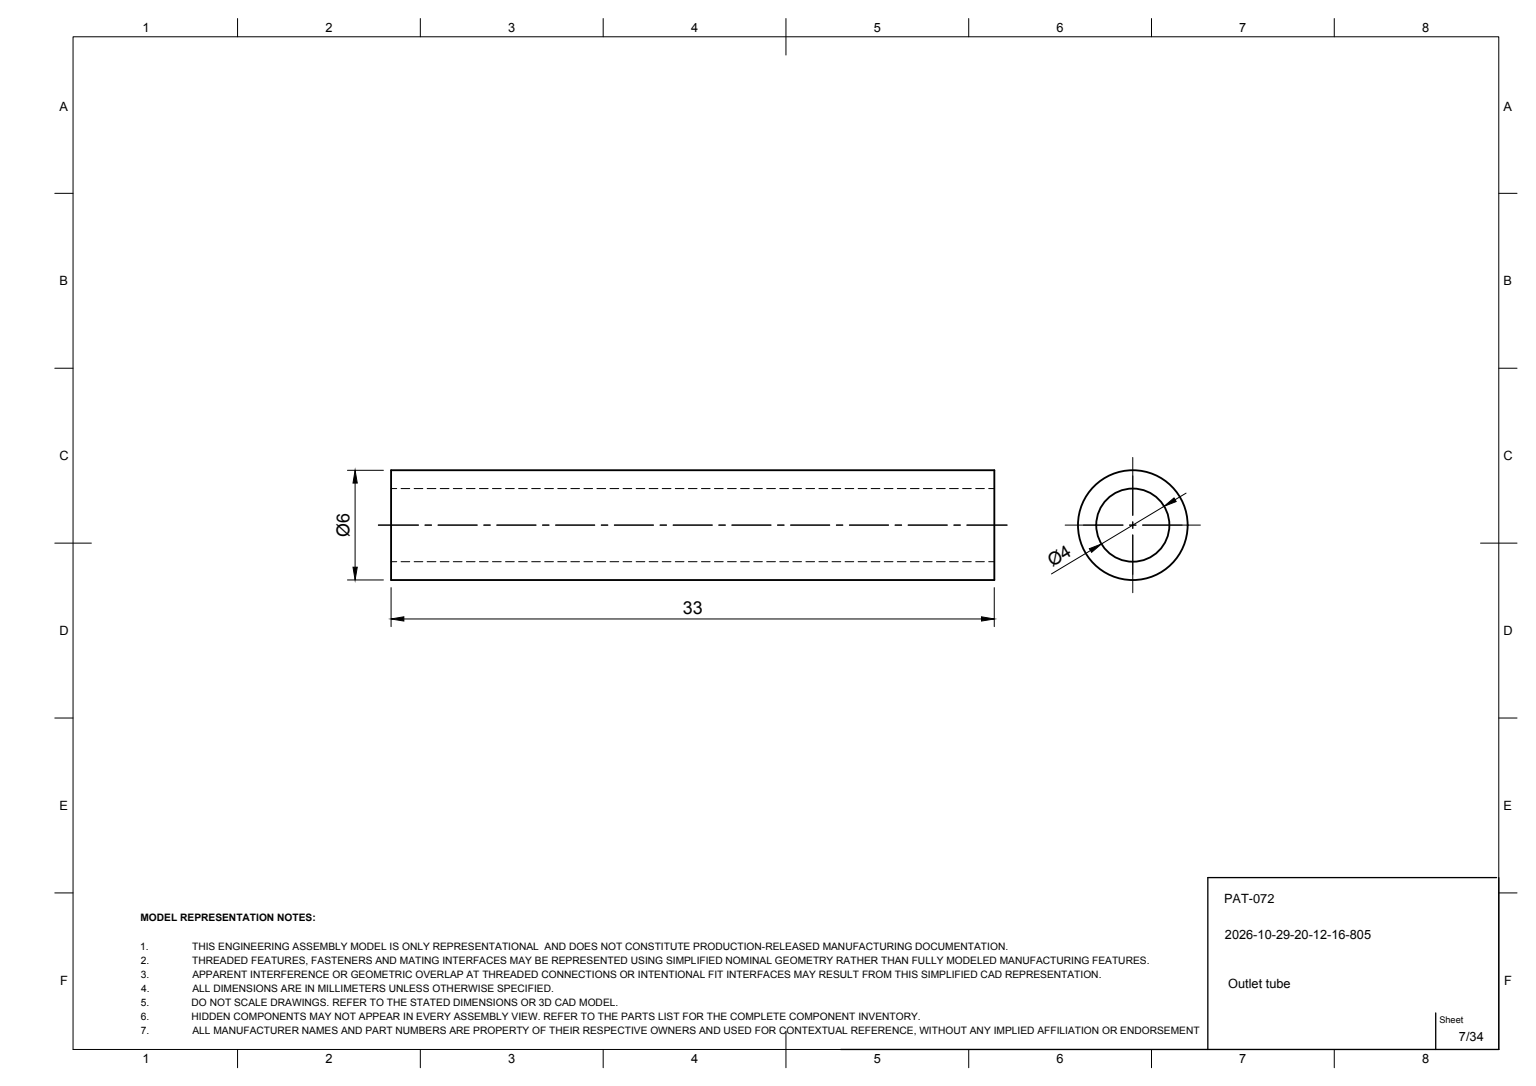
ISO-10303-21;
HEADER;
/* Generated by software containing ST-Developer
 * from STEP Tools, Inc. (www.steptools.com) 
 */

FILE_DESCRIPTION(
/* description */ ('PAT-072'),
/* implementation_level */ '2;1');

FILE_NAME(
/* name */ 'Outlet tube.step',
/* time_stamp */ '2026-10-29T20:11:56-07:00',
/* author */ (''),
/* organization */ (''),
/* preprocessor_version */ 'ST-DEVELOPER v20.2',
/* originating_system */ 'Autodesk Translation Framework v15.17.0.0',
/* authorisation */ '');

FILE_SCHEMA (('AUTOMOTIVE_DESIGN { 1 0 10303 214 3 1 1 }'));
ENDSEC;

DATA;
#10=MECHANICAL_DESIGN_GEOMETRIC_PRESENTATION_REPRESENTATION('',(#336),#11432);
#264=SHAPE_REPRESENTATION_RELATIONSHIP('SRR','None',#11568,#300);
#300=ADVANCED_BREP_SHAPE_REPRESENTATION('',(#372),#11399);
#336=STYLED_ITEM('',(#11812),#372);
#372=MANIFOLD_SOLID_BREP('Body1',#6071);
#460=FACE_BOUND('',#1326,.T.);
#461=FACE_BOUND('',#1328,.T.);
#621=PLANE('',#6699);
#622=PLANE('',#6700);
#893=FACE_OUTER_BOUND('',#1323,.T.);
#894=FACE_OUTER_BOUND('',#1324,.T.);
#895=FACE_OUTER_BOUND('',#1325,.T.);
#896=FACE_OUTER_BOUND('',#1327,.T.);
#1323=EDGE_LOOP('',(#4498,#4499,#4500,#4501));
#1324=EDGE_LOOP('',(#4502,#4503,#4504,#4505));
#1325=EDGE_LOOP('',(#4506));
#1326=EDGE_LOOP('',(#4507));
#1327=EDGE_LOOP('',(#4508));
#1328=EDGE_LOOP('',(#4509));
#1810=LINE('',#9993,#2229);
#1811=LINE('',#9999,#2230);
#2229=VECTOR('',#7747,0.2);
#2230=VECTOR('',#7754,0.3);
#2627=CIRCLE('',#6694,0.2);
#2628=CIRCLE('',#6695,0.2);
#2629=CIRCLE('',#6697,0.3);
#2630=CIRCLE('',#6698,0.3);
#2976=VERTEX_POINT('',#9990);
#2977=VERTEX_POINT('',#9992);
#2978=VERTEX_POINT('',#9996);
#2979=VERTEX_POINT('',#9998);
#3538=EDGE_CURVE('',#2976,#2976,#2627,.T.);
#3539=EDGE_CURVE('',#2976,#2977,#1810,.T.);
#3540=EDGE_CURVE('',#2977,#2977,#2628,.T.);
#3541=EDGE_CURVE('',#2978,#2978,#2629,.T.);
#3542=EDGE_CURVE('',#2978,#2979,#1811,.T.);
#3543=EDGE_CURVE('',#2979,#2979,#2630,.T.);
#4498=ORIENTED_EDGE('',*,*,#3538,.F.);
#4499=ORIENTED_EDGE('',*,*,#3539,.T.);
#4500=ORIENTED_EDGE('',*,*,#3540,.T.);
#4501=ORIENTED_EDGE('',*,*,#3539,.F.);
#4502=ORIENTED_EDGE('',*,*,#3541,.F.);
#4503=ORIENTED_EDGE('',*,*,#3542,.T.);
#4504=ORIENTED_EDGE('',*,*,#3543,.T.);
#4505=ORIENTED_EDGE('',*,*,#3542,.F.);
#4506=ORIENTED_EDGE('',*,*,#3541,.T.);
#4507=ORIENTED_EDGE('',*,*,#3538,.T.);
#4508=ORIENTED_EDGE('',*,*,#3543,.F.);
#4509=ORIENTED_EDGE('',*,*,#3540,.F.);
#5604=CYLINDRICAL_SURFACE('',#6693,0.2);
#5605=CYLINDRICAL_SURFACE('',#6696,0.3);
#5792=ADVANCED_FACE('',(#893),#5604,.F.);
#5793=ADVANCED_FACE('',(#894),#5605,.T.);
#5794=ADVANCED_FACE('',(#895,#460),#621,.T.);
#5795=ADVANCED_FACE('',(#896,#461),#622,.F.);
#6071=CLOSED_SHELL('',(#5792,#5793,#5794,#5795));
#6692=AXIS2_PLACEMENT_3D('',#9988,#7741,#7742);
#6693=AXIS2_PLACEMENT_3D('',#9989,#7743,#7744);
#6694=AXIS2_PLACEMENT_3D('',#9991,#7745,#7746);
#6695=AXIS2_PLACEMENT_3D('',#9994,#7748,#7749);
#6696=AXIS2_PLACEMENT_3D('',#9995,#7750,#7751);
#6697=AXIS2_PLACEMENT_3D('',#9997,#7752,#7753);
#6698=AXIS2_PLACEMENT_3D('',#10000,#7755,#7756);
#6699=AXIS2_PLACEMENT_3D('',#10001,#7757,#7758);
#6700=AXIS2_PLACEMENT_3D('',#10002,#7759,#7760);
#7741=DIRECTION('axis',(0.,0.,1.));
#7742=DIRECTION('refdir',(1.,0.,0.));
#7743=DIRECTION('center_axis',(0.,1.,0.));
#7744=DIRECTION('ref_axis',(1.,0.,0.));
#7745=DIRECTION('center_axis',(0.,-1.,0.));
#7746=DIRECTION('ref_axis',(1.,0.,0.));
#7747=DIRECTION('',(0.,-1.,0.));
#7748=DIRECTION('center_axis',(0.,-1.,0.));
#7749=DIRECTION('ref_axis',(1.,0.,0.));
#7750=DIRECTION('center_axis',(0.,1.,0.));
#7751=DIRECTION('ref_axis',(1.,0.,0.));
#7752=DIRECTION('center_axis',(0.,1.,0.));
#7753=DIRECTION('ref_axis',(1.,0.,0.));
#7754=DIRECTION('',(0.,-1.,0.));
#7755=DIRECTION('center_axis',(0.,1.,0.));
#7756=DIRECTION('ref_axis',(1.,0.,0.));
#7757=DIRECTION('center_axis',(0.,1.,0.));
#7758=DIRECTION('ref_axis',(1.,0.,0.));
#7759=DIRECTION('center_axis',(0.,1.,0.));
#7760=DIRECTION('ref_axis',(1.,0.,0.));
#9988=CARTESIAN_POINT('',(0.,0.,0.));
#9989=CARTESIAN_POINT('Origin',(-3.75,-6.5,4.));
#9990=CARTESIAN_POINT('',(-3.95,-3.2,4.));
#9991=CARTESIAN_POINT('Origin',(-3.75,-3.2,4.));
#9992=CARTESIAN_POINT('',(-3.95,-6.5,4.));
#9993=CARTESIAN_POINT('',(-3.95,-6.5,4.));
#9994=CARTESIAN_POINT('Origin',(-3.75,-6.5,4.));
#9995=CARTESIAN_POINT('Origin',(-3.75,-6.5,4.));
#9996=CARTESIAN_POINT('',(-4.05,-3.2,4.));
#9997=CARTESIAN_POINT('Origin',(-3.75,-3.2,4.));
#9998=CARTESIAN_POINT('',(-4.05,-6.5,4.));
#9999=CARTESIAN_POINT('',(-4.05,-6.5,4.));
#10000=CARTESIAN_POINT('Origin',(-3.75,-6.5,4.));
#10001=CARTESIAN_POINT('Origin',(-3.75,-3.2,4.));
#10002=CARTESIAN_POINT('Origin',(-3.75,-6.5,4.));
#11360=UNCERTAINTY_MEASURE_WITH_UNIT(LENGTH_MEASURE(0.001),#11433,
'DISTANCE_ACCURACY_VALUE',
'Maximum model space distance between geometric entities at asserted c
onnectivities');
#11393=UNCERTAINTY_MEASURE_WITH_UNIT(LENGTH_MEASURE(0.001),#11433,
'DISTANCE_ACCURACY_VALUE',
'Maximum model space distance between geometric entities at asserted c
onnectivities');
#11399=(
GEOMETRIC_REPRESENTATION_CONTEXT(3)
GLOBAL_UNCERTAINTY_ASSIGNED_CONTEXT((#11360))
GLOBAL_UNIT_ASSIGNED_CONTEXT((#11433,#11435,#11436))
REPRESENTATION_CONTEXT('','3D')
);
#11432=(
GEOMETRIC_REPRESENTATION_CONTEXT(3)
GLOBAL_UNCERTAINTY_ASSIGNED_CONTEXT((#11393))
GLOBAL_UNIT_ASSIGNED_CONTEXT((#11433,#11435,#11436))
REPRESENTATION_CONTEXT('','3D')
);
#11433=(
LENGTH_UNIT()
NAMED_UNIT(*)
SI_UNIT(.CENTI.,.METRE.)
);
#11435=(
NAMED_UNIT(*)
PLANE_ANGLE_UNIT()
SI_UNIT($,.RADIAN.)
);
#11436=(
NAMED_UNIT(*)
SI_UNIT($,.STERADIAN.)
SOLID_ANGLE_UNIT()
);
#11442=SHAPE_DEFINITION_REPRESENTATION(#11480,#11568);
#11480=PRODUCT_DEFINITION_SHAPE('',$,#11607);
#11568=SHAPE_REPRESENTATION('',(#6692),#11399);
#11601=PRODUCT_DEFINITION_CONTEXT('part definition',#11717,'design');
#11607=PRODUCT_DEFINITION('Outlet tube','Outlet tube',#11645,
#11601);
#11645=PRODUCT_DEFINITION_FORMATION('',$,#11724);
#11717=APPLICATION_CONTEXT(
'Core Data for Automotive Mechanical Design Process');
#11718=PRODUCT_CONTEXT('part definition',#11717,'mechanical');
#11724=PRODUCT('Outlet tube','Outlet tube','Outlet tube',(#11718));
#11806=COLOUR_RGB('Sky Blue',0.24,0.69,0.87);
#11807=FILL_AREA_STYLE_COLOUR('',#11806);
#11808=FILL_AREA_STYLE('',(#11807));
#11809=SURFACE_STYLE_FILL_AREA(#11808);
#11810=SURFACE_SIDE_STYLE('',(#11809));
#11811=SURFACE_STYLE_USAGE(.BOTH.,#11810);
#11812=PRESENTATION_STYLE_ASSIGNMENT((#11811));
ENDSEC;
END-ISO-10303-21;
